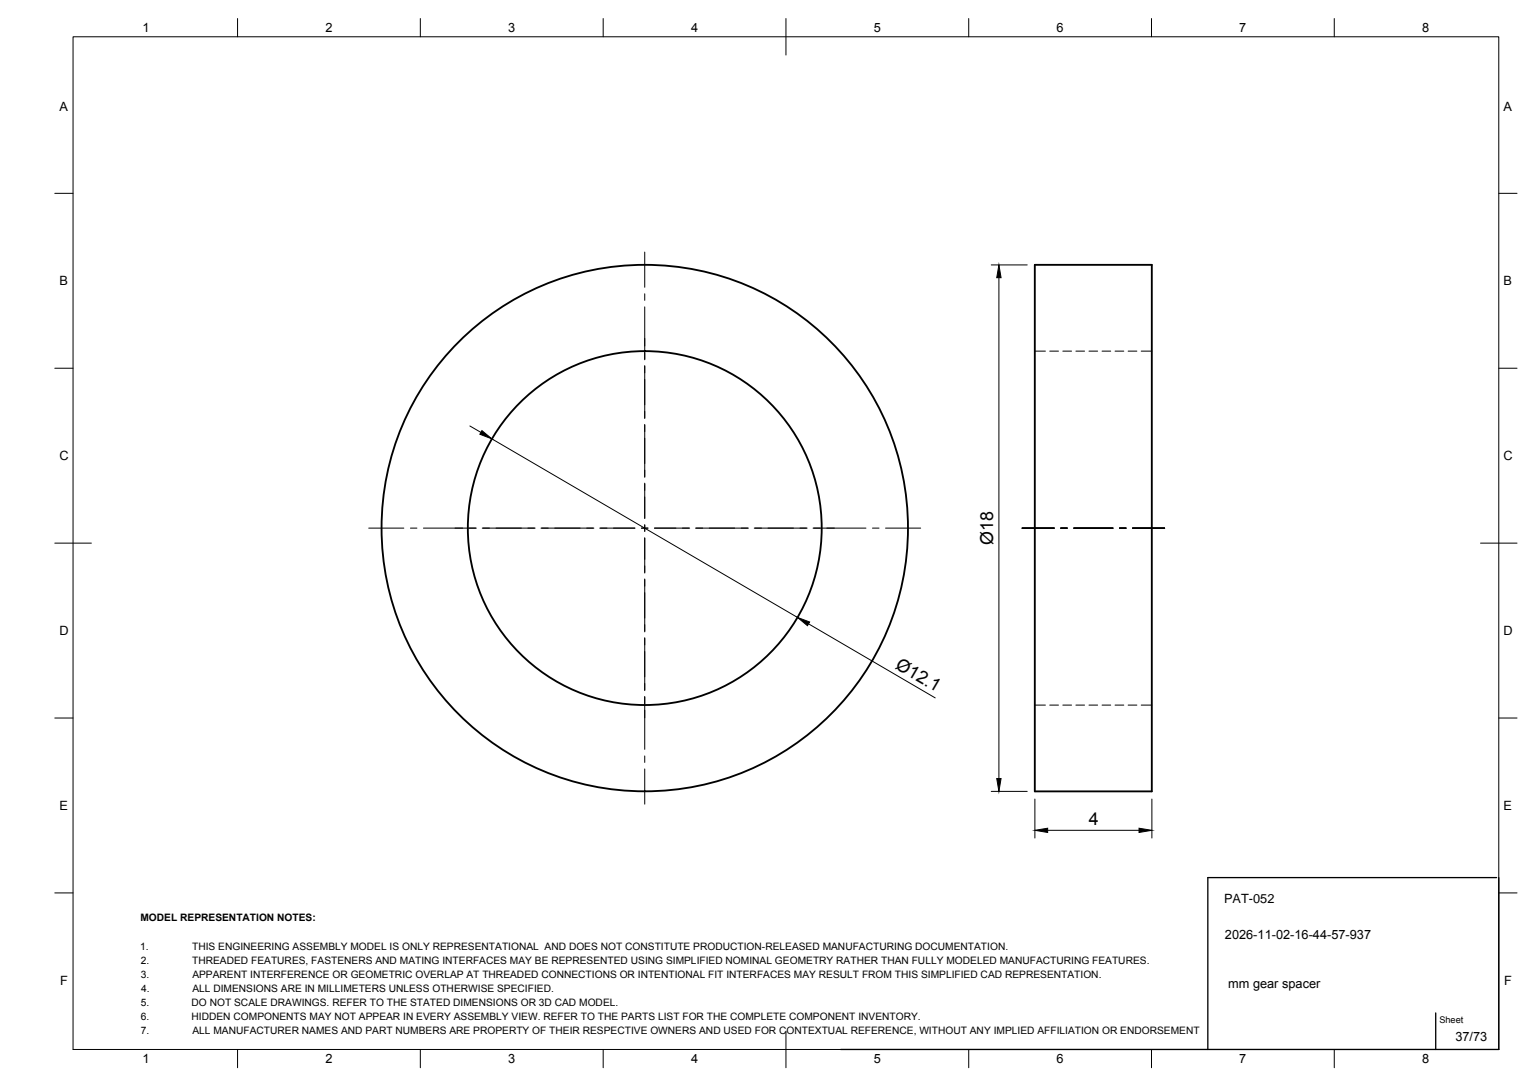
ISO-10303-21;
HEADER;
/* Generated by software containing ST-Developer
 * from STEP Tools, Inc. (www.steptools.com) 
 */

FILE_DESCRIPTION(
/* description */ ('Hand-crank gear train demonstrator'),
/* implementation_level */ '2;1');

FILE_NAME(
/* name */ 'mm gear spacer.step',
/* time_stamp */ '2026-10-28T03:22:13-07:00',
/* author */ (''),
/* organization */ (''),
/* preprocessor_version */ 'ST-DEVELOPER v20.2',
/* originating_system */ 'Autodesk Translation Framework v15.17.0.0',
/* authorisation */ '');

FILE_SCHEMA (('AUTOMOTIVE_DESIGN { 1 0 10303 214 3 1 1 }'));
ENDSEC;

DATA;
#10=MECHANICAL_DESIGN_GEOMETRIC_PRESENTATION_REPRESENTATION('',(#1233),#62758);
#1090=SHAPE_REPRESENTATION_RELATIONSHIP('SRR','None',#63065,#1154);
#1154=ADVANCED_BREP_SHAPE_REPRESENTATION('',(#1309),#62719);
#1233=STYLED_ITEM('',(#63476),#1309);
#1309=MANIFOLD_SOLID_BREP('Body1',#16416);
#1547=FACE_BOUND('',#3710,.T.);
#1548=FACE_BOUND('',#3712,.T.);
#1898=PLANE('',#18012);
#1899=PLANE('',#18013);
#2566=FACE_OUTER_BOUND('',#3707,.T.);
#2567=FACE_OUTER_BOUND('',#3708,.T.);
#2568=FACE_OUTER_BOUND('',#3709,.T.);
#2569=FACE_OUTER_BOUND('',#3711,.T.);
#3707=EDGE_LOOP('',(#12781,#12782,#12783,#12784));
#3708=EDGE_LOOP('',(#12785,#12786,#12787,#12788));
#3709=EDGE_LOOP('',(#12789));
#3710=EDGE_LOOP('',(#12790));
#3711=EDGE_LOOP('',(#12791));
#3712=EDGE_LOOP('',(#12792));
#4867=LINE('',#26069,#5999);
#4868=LINE('',#26075,#6000);
#5999=VECTOR('',#21112,0.605);
#6000=VECTOR('',#21119,0.9);
#6910=CIRCLE('',#18007,0.605);
#6911=CIRCLE('',#18008,0.605);
#6912=CIRCLE('',#18010,0.9);
#6913=CIRCLE('',#18011,0.9);
#7875=VERTEX_POINT('',#26066);
#7876=VERTEX_POINT('',#26068);
#7877=VERTEX_POINT('',#26072);
#7878=VERTEX_POINT('',#26074);
#9642=EDGE_CURVE('',#7875,#7875,#6910,.T.);
#9643=EDGE_CURVE('',#7875,#7876,#4867,.T.);
#9644=EDGE_CURVE('',#7876,#7876,#6911,.T.);
#9645=EDGE_CURVE('',#7877,#7877,#6912,.T.);
#9646=EDGE_CURVE('',#7877,#7878,#4868,.T.);
#9647=EDGE_CURVE('',#7878,#7878,#6913,.T.);
#12781=ORIENTED_EDGE('',*,*,#9642,.F.);
#12782=ORIENTED_EDGE('',*,*,#9643,.T.);
#12783=ORIENTED_EDGE('',*,*,#9644,.T.);
#12784=ORIENTED_EDGE('',*,*,#9643,.F.);
#12785=ORIENTED_EDGE('',*,*,#9645,.F.);
#12786=ORIENTED_EDGE('',*,*,#9646,.T.);
#12787=ORIENTED_EDGE('',*,*,#9647,.T.);
#12788=ORIENTED_EDGE('',*,*,#9646,.F.);
#12789=ORIENTED_EDGE('',*,*,#9645,.T.);
#12790=ORIENTED_EDGE('',*,*,#9642,.T.);
#12791=ORIENTED_EDGE('',*,*,#9647,.F.);
#12792=ORIENTED_EDGE('',*,*,#9644,.F.);
#15294=CYLINDRICAL_SURFACE('',#18006,0.605);
#15295=CYLINDRICAL_SURFACE('',#18009,0.9);
#15876=ADVANCED_FACE('',(#2566),#15294,.F.);
#15877=ADVANCED_FACE('',(#2567),#15295,.T.);
#15878=ADVANCED_FACE('',(#2568,#1547),#1898,.T.);
#15879=ADVANCED_FACE('',(#2569,#1548),#1899,.F.);
#16416=CLOSED_SHELL('',(#15876,#15877,#15878,#15879));
#18005=AXIS2_PLACEMENT_3D('',#26064,#21106,#21107);
#18006=AXIS2_PLACEMENT_3D('',#26065,#21108,#21109);
#18007=AXIS2_PLACEMENT_3D('',#26067,#21110,#21111);
#18008=AXIS2_PLACEMENT_3D('',#26070,#21113,#21114);
#18009=AXIS2_PLACEMENT_3D('',#26071,#21115,#21116);
#18010=AXIS2_PLACEMENT_3D('',#26073,#21117,#21118);
#18011=AXIS2_PLACEMENT_3D('',#26076,#21120,#21121);
#18012=AXIS2_PLACEMENT_3D('',#26077,#21122,#21123);
#18013=AXIS2_PLACEMENT_3D('',#26078,#21124,#21125);
#21106=DIRECTION('axis',(0.,0.,1.));
#21107=DIRECTION('refdir',(1.,0.,0.));
#21108=DIRECTION('center_axis',(0.,1.,0.));
#21109=DIRECTION('ref_axis',(1.,0.,0.));
#21110=DIRECTION('center_axis',(0.,-1.,0.));
#21111=DIRECTION('ref_axis',(1.,0.,0.));
#21112=DIRECTION('',(0.,-1.,0.));
#21113=DIRECTION('center_axis',(0.,-1.,0.));
#21114=DIRECTION('ref_axis',(1.,0.,0.));
#21115=DIRECTION('center_axis',(0.,1.,0.));
#21116=DIRECTION('ref_axis',(1.,0.,0.));
#21117=DIRECTION('center_axis',(0.,1.,0.));
#21118=DIRECTION('ref_axis',(1.,0.,0.));
#21119=DIRECTION('',(0.,-1.,0.));
#21120=DIRECTION('center_axis',(0.,1.,0.));
#21121=DIRECTION('ref_axis',(1.,0.,0.));
#21122=DIRECTION('center_axis',(0.,1.,0.));
#21123=DIRECTION('ref_axis',(1.,0.,0.));
#21124=DIRECTION('center_axis',(0.,1.,0.));
#21125=DIRECTION('ref_axis',(1.,0.,0.));
#26064=CARTESIAN_POINT('',(0.,0.,0.));
#26065=CARTESIAN_POINT('Origin',(0.,-0.4,9.));
#26066=CARTESIAN_POINT('',(-0.605,0.,9.));
#26067=CARTESIAN_POINT('Origin',(0.,0.,9.));
#26068=CARTESIAN_POINT('',(-0.605,-0.4,9.));
#26069=CARTESIAN_POINT('',(-0.605,-0.4,9.));
#26070=CARTESIAN_POINT('Origin',(0.,-0.4,9.));
#26071=CARTESIAN_POINT('Origin',(0.,-0.4,9.));
#26072=CARTESIAN_POINT('',(-0.9,0.,9.));
#26073=CARTESIAN_POINT('Origin',(0.,0.,9.));
#26074=CARTESIAN_POINT('',(-0.9,-0.4,9.));
#26075=CARTESIAN_POINT('',(-0.9,-0.4,9.));
#26076=CARTESIAN_POINT('Origin',(0.,-0.4,9.));
#26077=CARTESIAN_POINT('Origin',(0.,0.,9.));
#26078=CARTESIAN_POINT('Origin',(0.,-0.4,9.));
#62645=UNCERTAINTY_MEASURE_WITH_UNIT(LENGTH_MEASURE(0.001),#62759,
'DISTANCE_ACCURACY_VALUE',
'Maximum model space distance between geometric entities at asserted c
onnectivities');
#62684=UNCERTAINTY_MEASURE_WITH_UNIT(LENGTH_MEASURE(0.001),#62759,
'DISTANCE_ACCURACY_VALUE',
'Maximum model space distance between geometric entities at asserted c
onnectivities');
#62719=(
GEOMETRIC_REPRESENTATION_CONTEXT(3)
GLOBAL_UNCERTAINTY_ASSIGNED_CONTEXT((#62645))
GLOBAL_UNIT_ASSIGNED_CONTEXT((#62759,#62761,#62762))
REPRESENTATION_CONTEXT('','3D')
);
#62758=(
GEOMETRIC_REPRESENTATION_CONTEXT(3)
GLOBAL_UNCERTAINTY_ASSIGNED_CONTEXT((#62684))
GLOBAL_UNIT_ASSIGNED_CONTEXT((#62759,#62761,#62762))
REPRESENTATION_CONTEXT('','3D')
);
#62759=(
LENGTH_UNIT()
NAMED_UNIT(*)
SI_UNIT(.CENTI.,.METRE.)
);
#62761=(
NAMED_UNIT(*)
PLANE_ANGLE_UNIT()
SI_UNIT($,.RADIAN.)
);
#62762=(
NAMED_UNIT(*)
SI_UNIT($,.STERADIAN.)
SOLID_ANGLE_UNIT()
);
#62797=SHAPE_DEFINITION_REPRESENTATION(#62880,#63065);
#62880=PRODUCT_DEFINITION_SHAPE('',$,#63139);
#63065=SHAPE_REPRESENTATION('',(#18005),#62719);
#63104=PRODUCT_DEFINITION_CONTEXT('part definition',#63325,'design');
#63139=PRODUCT_DEFINITION('mm gear spacer','mm gear spacer',#63212,#63104);
#63212=PRODUCT_DEFINITION_FORMATION('',$,#63361);
#63325=APPLICATION_CONTEXT(
'Core Data for Automotive Mechanical Design Process');
#63326=PRODUCT_CONTEXT('part definition',#63325,'mechanical');
#63361=PRODUCT('mm gear spacer','mm gear spacer','mm gear spacer',(#63326));
#63470=COLOUR_RGB('Off White',0.89,0.88,0.83);
#63471=FILL_AREA_STYLE_COLOUR('',#63470);
#63472=FILL_AREA_STYLE('',(#63471));
#63473=SURFACE_STYLE_FILL_AREA(#63472);
#63474=SURFACE_SIDE_STYLE('',(#63473));
#63475=SURFACE_STYLE_USAGE(.BOTH.,#63474);
#63476=PRESENTATION_STYLE_ASSIGNMENT((#63475));
ENDSEC;
END-ISO-10303-21;
